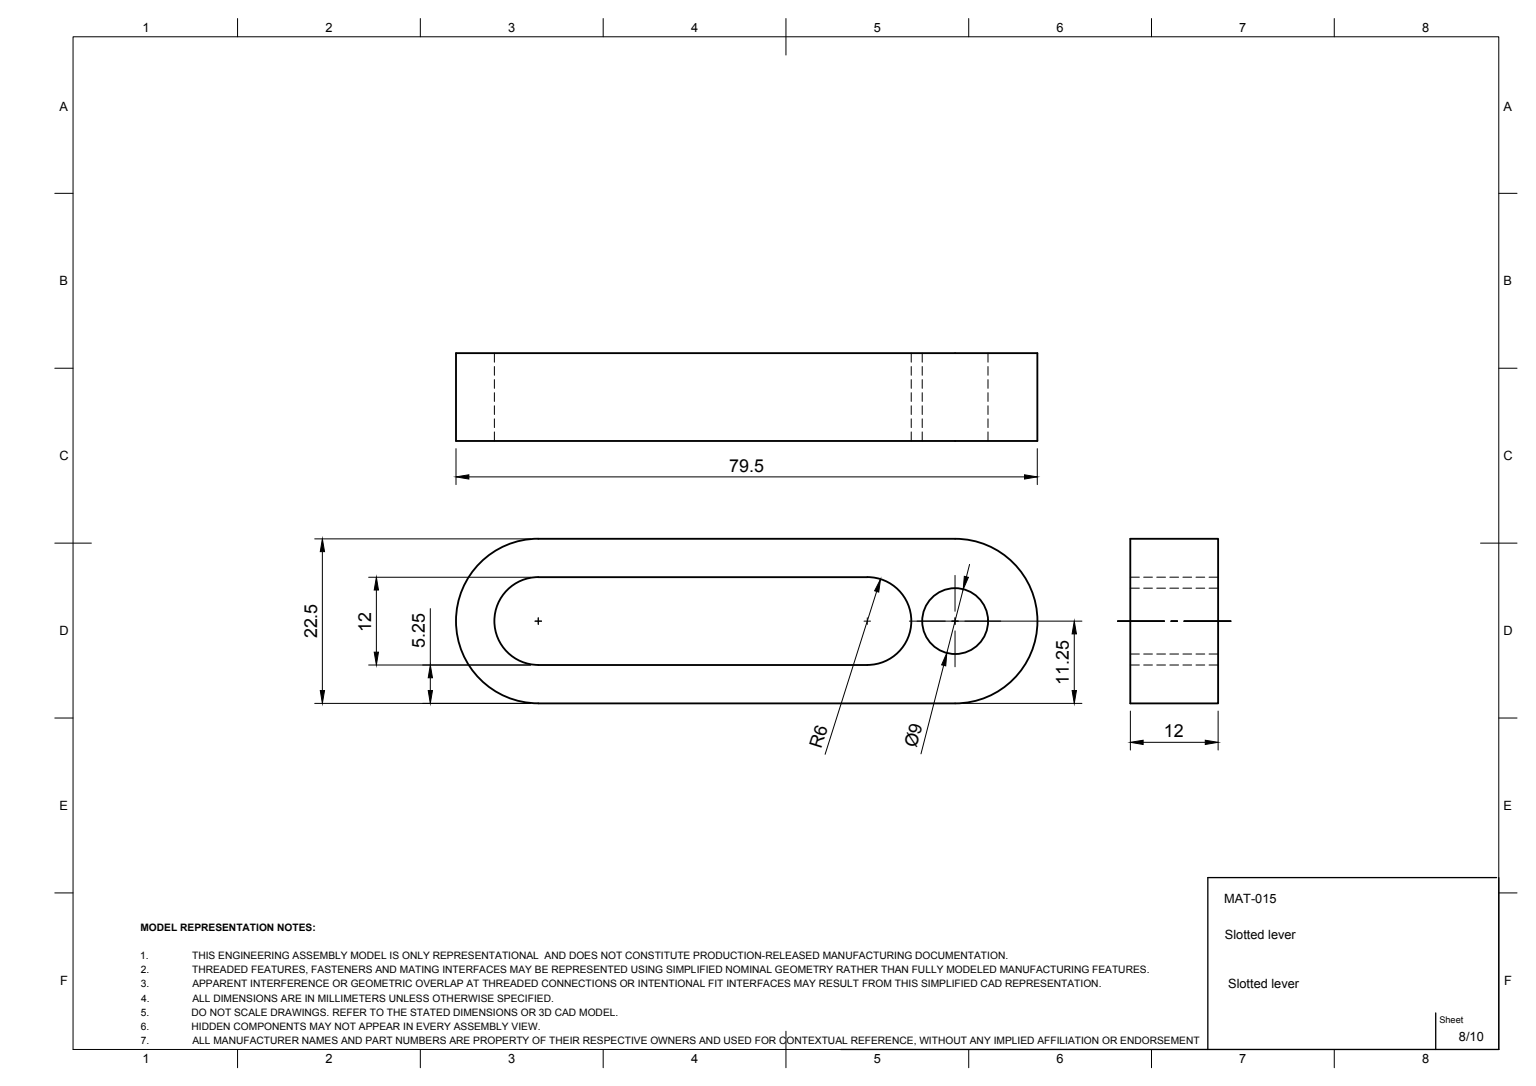
ISO-10303-21;
HEADER;
/* Generated by software containing ST-Developer
 * from STEP Tools, Inc. (www.steptools.com) 
 */

FILE_DESCRIPTION(
/* description */ ('STEP AP214'),
/* implementation_level */ '2;1');

FILE_NAME(
/* name */ 'Slotted Lever.step',
/* time_stamp */ '2026-11-14T06:03:18-08:00',
/* author */ (''),
/* organization */ (''),
/* preprocessor_version */ 'ST-DEVELOPER v20.2',
/* originating_system */ 'Autodesk Translation Framework v15.17.0.0',
/* authorisation */ '');

FILE_SCHEMA (('AUTOMOTIVE_DESIGN { 1 0 10303 214 3 1 1 }'));
ENDSEC;

DATA;
#10=MECHANICAL_DESIGN_GEOMETRIC_PRESENTATION_REPRESENTATION('',(#76),#3206);
#60=SHAPE_REPRESENTATION_RELATIONSHIP('SRR','None',#3243,#68);
#68=ADVANCED_BREP_SHAPE_REPRESENTATION('',(#84),#3202);
#76=STYLED_ITEM('',(#3288),#84);
#84=MANIFOLD_SOLID_BREP('Body1',#1783);
#111=PLANE('',#1971);
#112=PLANE('',#1974);
#113=PLANE('',#1978);
#114=PLANE('',#1979);
#115=PLANE('',#1981);
#116=PLANE('',#1982);
#164=FACE_BOUND('',#675,.T.);
#165=FACE_BOUND('',#676,.T.);
#166=FACE_BOUND('',#678,.T.);
#167=FACE_BOUND('',#679,.T.);
#227=LINE('',#2874,#372);
#228=LINE('',#2877,#373);
#229=LINE('',#2882,#374);
#230=LINE('',#2889,#375);
#231=LINE('',#2892,#376);
#232=LINE('',#2897,#377);
#233=LINE('',#2898,#378);
#234=LINE('',#2902,#379);
#235=LINE('',#2903,#380);
#236=LINE('',#2908,#381);
#237=LINE('',#2909,#382);
#238=LINE('',#2911,#383);
#239=LINE('',#2914,#384);
#240=LINE('',#2916,#385);
#241=LINE('',#2917,#386);
#242=LINE('',#2921,#387);
#243=LINE('',#2922,#388);
#372=VECTOR('',#2290,1000.);
#373=VECTOR('',#2293,1000.);
#374=VECTOR('',#2298,4.5);
#375=VECTOR('',#2305,1000.);
#376=VECTOR('',#2308,1000.);
#377=VECTOR('',#2313,1000.);
#378=VECTOR('',#2314,1000.);
#379=VECTOR('',#2317,1000.);
#380=VECTOR('',#2318,1000.);
#381=VECTOR('',#2323,1000.);
#382=VECTOR('',#2324,1000.);
#383=VECTOR('',#2325,1000.);
#384=VECTOR('',#2328,1000.);
#385=VECTOR('',#2331,1000.);
#386=VECTOR('',#2332,1000.);
#387=VECTOR('',#2339,1000.);
#388=VECTOR('',#2340,1000.);
#492=CYLINDRICAL_SURFACE('',#1962,6.);
#493=CYLINDRICAL_SURFACE('',#1965,4.5);
#494=CYLINDRICAL_SURFACE('',#1968,11.25);
#495=CYLINDRICAL_SURFACE('',#1977,11.25);
#496=CYLINDRICAL_SURFACE('',#1980,6.);
#554=FACE_OUTER_BOUND('',#671,.T.);
#555=FACE_OUTER_BOUND('',#672,.T.);
#556=FACE_OUTER_BOUND('',#673,.T.);
#557=FACE_OUTER_BOUND('',#674,.T.);
#558=FACE_OUTER_BOUND('',#677,.T.);
#559=FACE_OUTER_BOUND('',#680,.T.);
#560=FACE_OUTER_BOUND('',#681,.T.);
#561=FACE_OUTER_BOUND('',#682,.T.);
#562=FACE_OUTER_BOUND('',#683,.T.);
#563=FACE_OUTER_BOUND('',#684,.T.);
#564=FACE_OUTER_BOUND('',#685,.T.);
#671=EDGE_LOOP('',(#1379,#1380,#1381,#1382));
#672=EDGE_LOOP('',(#1383,#1384,#1385,#1386));
#673=EDGE_LOOP('',(#1387,#1388,#1389,#1390));
#674=EDGE_LOOP('',(#1391,#1392,#1393,#1394));
#675=EDGE_LOOP('',(#1395,#1396,#1397,#1398));
#676=EDGE_LOOP('',(#1399));
#677=EDGE_LOOP('',(#1400,#1401,#1402,#1403));
#678=EDGE_LOOP('',(#1404,#1405,#1406,#1407));
#679=EDGE_LOOP('',(#1408));
#680=EDGE_LOOP('',(#1409,#1410,#1411,#1412));
#681=EDGE_LOOP('',(#1413,#1414,#1415,#1416));
#682=EDGE_LOOP('',(#1417,#1418,#1419,#1420));
#683=EDGE_LOOP('',(#1421,#1422,#1423,#1424));
#684=EDGE_LOOP('',(#1425,#1426,#1427,#1428));
#685=EDGE_LOOP('',(#1429,#1430,#1431,#1432));
#791=CIRCLE('',#1963,6.);
#792=CIRCLE('',#1964,6.);
#793=CIRCLE('',#1966,4.5);
#794=CIRCLE('',#1967,4.5);
#795=CIRCLE('',#1969,11.25);
#796=CIRCLE('',#1970,11.25);
#797=CIRCLE('',#1972,11.25);
#798=CIRCLE('',#1973,6.);
#799=CIRCLE('',#1975,11.25);
#800=CIRCLE('',#1976,6.);
#888=VERTEX_POINT('',#2870);
#889=VERTEX_POINT('',#2871);
#890=VERTEX_POINT('',#2873);
#891=VERTEX_POINT('',#2875);
#892=VERTEX_POINT('',#2879);
#893=VERTEX_POINT('',#2881);
#894=VERTEX_POINT('',#2885);
#895=VERTEX_POINT('',#2886);
#896=VERTEX_POINT('',#2888);
#897=VERTEX_POINT('',#2890);
#898=VERTEX_POINT('',#2894);
#899=VERTEX_POINT('',#2895);
#900=VERTEX_POINT('',#2899);
#901=VERTEX_POINT('',#2900);
#902=VERTEX_POINT('',#2905);
#903=VERTEX_POINT('',#2906);
#904=VERTEX_POINT('',#2910);
#905=VERTEX_POINT('',#2912);
#1068=EDGE_CURVE('',#888,#889,#791,.T.);
#1069=EDGE_CURVE('',#889,#890,#227,.T.);
#1070=EDGE_CURVE('',#891,#890,#792,.T.);
#1071=EDGE_CURVE('',#888,#891,#228,.T.);
#1072=EDGE_CURVE('',#892,#892,#793,.T.);
#1073=EDGE_CURVE('',#892,#893,#229,.T.);
#1074=EDGE_CURVE('',#893,#893,#794,.T.);
#1075=EDGE_CURVE('',#894,#895,#795,.T.);
#1076=EDGE_CURVE('',#894,#896,#230,.T.);
#1077=EDGE_CURVE('',#896,#897,#796,.T.);
#1078=EDGE_CURVE('',#895,#897,#231,.T.);
#1079=EDGE_CURVE('',#898,#899,#797,.T.);
#1080=EDGE_CURVE('',#899,#894,#232,.T.);
#1081=EDGE_CURVE('',#895,#898,#233,.T.);
#1082=EDGE_CURVE('',#900,#901,#798,.T.);
#1083=EDGE_CURVE('',#889,#900,#234,.T.);
#1084=EDGE_CURVE('',#901,#888,#235,.T.);
#1085=EDGE_CURVE('',#902,#903,#799,.T.);
#1086=EDGE_CURVE('',#897,#902,#236,.T.);
#1087=EDGE_CURVE('',#903,#896,#237,.T.);
#1088=EDGE_CURVE('',#890,#904,#238,.T.);
#1089=EDGE_CURVE('',#904,#905,#800,.T.);
#1090=EDGE_CURVE('',#905,#891,#239,.T.);
#1091=EDGE_CURVE('',#899,#903,#240,.T.);
#1092=EDGE_CURVE('',#898,#902,#241,.T.);
#1093=EDGE_CURVE('',#900,#904,#242,.T.);
#1094=EDGE_CURVE('',#901,#905,#243,.T.);
#1379=ORIENTED_EDGE('',*,*,#1068,.T.);
#1380=ORIENTED_EDGE('',*,*,#1069,.T.);
#1381=ORIENTED_EDGE('',*,*,#1070,.F.);
#1382=ORIENTED_EDGE('',*,*,#1071,.F.);
#1383=ORIENTED_EDGE('',*,*,#1072,.T.);
#1384=ORIENTED_EDGE('',*,*,#1073,.T.);
#1385=ORIENTED_EDGE('',*,*,#1074,.F.);
#1386=ORIENTED_EDGE('',*,*,#1073,.F.);
#1387=ORIENTED_EDGE('',*,*,#1075,.F.);
#1388=ORIENTED_EDGE('',*,*,#1076,.T.);
#1389=ORIENTED_EDGE('',*,*,#1077,.T.);
#1390=ORIENTED_EDGE('',*,*,#1078,.F.);
#1391=ORIENTED_EDGE('',*,*,#1079,.T.);
#1392=ORIENTED_EDGE('',*,*,#1080,.T.);
#1393=ORIENTED_EDGE('',*,*,#1075,.T.);
#1394=ORIENTED_EDGE('',*,*,#1081,.T.);
#1395=ORIENTED_EDGE('',*,*,#1082,.F.);
#1396=ORIENTED_EDGE('',*,*,#1083,.F.);
#1397=ORIENTED_EDGE('',*,*,#1068,.F.);
#1398=ORIENTED_EDGE('',*,*,#1084,.F.);
#1399=ORIENTED_EDGE('',*,*,#1072,.F.);
#1400=ORIENTED_EDGE('',*,*,#1085,.F.);
#1401=ORIENTED_EDGE('',*,*,#1086,.F.);
#1402=ORIENTED_EDGE('',*,*,#1077,.F.);
#1403=ORIENTED_EDGE('',*,*,#1087,.F.);
#1404=ORIENTED_EDGE('',*,*,#1088,.T.);
#1405=ORIENTED_EDGE('',*,*,#1089,.T.);
#1406=ORIENTED_EDGE('',*,*,#1090,.T.);
#1407=ORIENTED_EDGE('',*,*,#1070,.T.);
#1408=ORIENTED_EDGE('',*,*,#1074,.T.);
#1409=ORIENTED_EDGE('',*,*,#1085,.T.);
#1410=ORIENTED_EDGE('',*,*,#1091,.F.);
#1411=ORIENTED_EDGE('',*,*,#1079,.F.);
#1412=ORIENTED_EDGE('',*,*,#1092,.T.);
#1413=ORIENTED_EDGE('',*,*,#1087,.T.);
#1414=ORIENTED_EDGE('',*,*,#1076,.F.);
#1415=ORIENTED_EDGE('',*,*,#1080,.F.);
#1416=ORIENTED_EDGE('',*,*,#1091,.T.);
#1417=ORIENTED_EDGE('',*,*,#1086,.T.);
#1418=ORIENTED_EDGE('',*,*,#1092,.F.);
#1419=ORIENTED_EDGE('',*,*,#1081,.F.);
#1420=ORIENTED_EDGE('',*,*,#1078,.T.);
#1421=ORIENTED_EDGE('',*,*,#1089,.F.);
#1422=ORIENTED_EDGE('',*,*,#1093,.F.);
#1423=ORIENTED_EDGE('',*,*,#1082,.T.);
#1424=ORIENTED_EDGE('',*,*,#1094,.T.);
#1425=ORIENTED_EDGE('',*,*,#1090,.F.);
#1426=ORIENTED_EDGE('',*,*,#1094,.F.);
#1427=ORIENTED_EDGE('',*,*,#1084,.T.);
#1428=ORIENTED_EDGE('',*,*,#1071,.T.);
#1429=ORIENTED_EDGE('',*,*,#1088,.F.);
#1430=ORIENTED_EDGE('',*,*,#1069,.F.);
#1431=ORIENTED_EDGE('',*,*,#1083,.T.);
#1432=ORIENTED_EDGE('',*,*,#1093,.T.);
#1721=ADVANCED_FACE('',(#554),#492,.F.);
#1722=ADVANCED_FACE('',(#555),#493,.F.);
#1723=ADVANCED_FACE('',(#556),#494,.T.);
#1724=ADVANCED_FACE('',(#557,#164,#165),#111,.F.);
#1725=ADVANCED_FACE('',(#558,#166,#167),#112,.T.);
#1726=ADVANCED_FACE('',(#559),#495,.T.);
#1727=ADVANCED_FACE('',(#560),#113,.F.);
#1728=ADVANCED_FACE('',(#561),#114,.F.);
#1729=ADVANCED_FACE('',(#562),#496,.F.);
#1730=ADVANCED_FACE('',(#563),#115,.T.);
#1731=ADVANCED_FACE('',(#564),#116,.T.);
#1783=CLOSED_SHELL('',(#1721,#1722,#1723,#1724,#1725,#1726,#1727,#1728,
#1729,#1730,#1731));
#1961=AXIS2_PLACEMENT_3D('',#2868,#2284,#2285);
#1962=AXIS2_PLACEMENT_3D('',#2869,#2286,#2287);
#1963=AXIS2_PLACEMENT_3D('',#2872,#2288,#2289);
#1964=AXIS2_PLACEMENT_3D('',#2876,#2291,#2292);
#1965=AXIS2_PLACEMENT_3D('',#2878,#2294,#2295);
#1966=AXIS2_PLACEMENT_3D('',#2880,#2296,#2297);
#1967=AXIS2_PLACEMENT_3D('',#2883,#2299,#2300);
#1968=AXIS2_PLACEMENT_3D('',#2884,#2301,#2302);
#1969=AXIS2_PLACEMENT_3D('',#2887,#2303,#2304);
#1970=AXIS2_PLACEMENT_3D('',#2891,#2306,#2307);
#1971=AXIS2_PLACEMENT_3D('',#2893,#2309,#2310);
#1972=AXIS2_PLACEMENT_3D('',#2896,#2311,#2312);
#1973=AXIS2_PLACEMENT_3D('',#2901,#2315,#2316);
#1974=AXIS2_PLACEMENT_3D('',#2904,#2319,#2320);
#1975=AXIS2_PLACEMENT_3D('',#2907,#2321,#2322);
#1976=AXIS2_PLACEMENT_3D('',#2913,#2326,#2327);
#1977=AXIS2_PLACEMENT_3D('',#2915,#2329,#2330);
#1978=AXIS2_PLACEMENT_3D('',#2918,#2333,#2334);
#1979=AXIS2_PLACEMENT_3D('',#2919,#2335,#2336);
#1980=AXIS2_PLACEMENT_3D('',#2920,#2337,#2338);
#1981=AXIS2_PLACEMENT_3D('',#2923,#2341,#2342);
#1982=AXIS2_PLACEMENT_3D('',#2924,#2343,#2344);
#2284=DIRECTION('axis',(0.,0.,1.));
#2285=DIRECTION('refdir',(1.,0.,0.));
#2286=DIRECTION('center_axis',(-1.15555796663234E-33,0.,-1.));
#2287=DIRECTION('ref_axis',(-1.,0.,1.15555796663234E-33));
#2288=DIRECTION('center_axis',(1.15555796663234E-33,0.,1.));
#2289=DIRECTION('ref_axis',(1.,0.,-1.15555796663234E-33));
#2290=DIRECTION('',(-1.15555796663234E-33,0.,-1.));
#2291=DIRECTION('center_axis',(1.15555796663234E-33,0.,1.));
#2292=DIRECTION('ref_axis',(1.,0.,-1.15555796663234E-33));
#2293=DIRECTION('',(-1.15555796663234E-33,0.,-1.));
#2294=DIRECTION('center_axis',(-1.15555796663234E-33,0.,-1.));
#2295=DIRECTION('ref_axis',(-1.,0.,1.15555796663234E-33));
#2296=DIRECTION('center_axis',(1.15555796663234E-33,0.,1.));
#2297=DIRECTION('ref_axis',(1.,0.,-1.15555796663234E-33));
#2298=DIRECTION('',(-1.15555796663234E-33,0.,-1.));
#2299=DIRECTION('center_axis',(1.15555796663234E-33,0.,1.));
#2300=DIRECTION('ref_axis',(1.,0.,-1.15555796663234E-33));
#2301=DIRECTION('center_axis',(-1.15555796663234E-33,0.,-1.));
#2302=DIRECTION('ref_axis',(-1.,0.,1.15555796663234E-33));
#2303=DIRECTION('center_axis',(1.15555796663234E-33,0.,1.));
#2304=DIRECTION('ref_axis',(1.,0.,-1.15555796663234E-33));
#2305=DIRECTION('',(-1.15555796663234E-33,0.,-1.));
#2306=DIRECTION('center_axis',(1.15555796663234E-33,0.,1.));
#2307=DIRECTION('ref_axis',(1.,0.,-1.15555796663234E-33));
#2308=DIRECTION('',(-1.15555796663234E-33,0.,-1.));
#2309=DIRECTION('center_axis',(1.15555796663234E-33,0.,-1.));
#2310=DIRECTION('ref_axis',(-1.,0.,-1.15555796663234E-33));
#2311=DIRECTION('center_axis',(1.15555796663234E-33,0.,1.));
#2312=DIRECTION('ref_axis',(-1.,0.,1.15555796663234E-33));
#2313=DIRECTION('',(-1.,0.,-1.15555796663234E-33));
#2314=DIRECTION('',(1.,0.,1.15555796663234E-33));
#2315=DIRECTION('center_axis',(1.15555796663234E-33,0.,1.));
#2316=DIRECTION('ref_axis',(1.,0.,-1.15555796663234E-33));
#2317=DIRECTION('',(1.,0.,1.15555796663234E-33));
#2318=DIRECTION('',(-1.,0.,-1.15555796663234E-33));
#2319=DIRECTION('center_axis',(1.15555796663234E-33,0.,-1.));
#2320=DIRECTION('ref_axis',(-1.,0.,-1.15555796663234E-33));
#2321=DIRECTION('center_axis',(1.15555796663234E-33,0.,1.));
#2322=DIRECTION('ref_axis',(-1.,0.,1.15555796663234E-33));
#2323=DIRECTION('',(1.,0.,1.15555796663234E-33));
#2324=DIRECTION('',(-1.,0.,-1.15555796663234E-33));
#2325=DIRECTION('',(1.,0.,1.15555796663234E-33));
#2326=DIRECTION('center_axis',(1.15555796663234E-33,0.,1.));
#2327=DIRECTION('ref_axis',(1.,0.,-1.15555796663234E-33));
#2328=DIRECTION('',(-1.,0.,-1.15555796663234E-33));
#2329=DIRECTION('center_axis',(-1.15555796663234E-33,0.,-1.));
#2330=DIRECTION('ref_axis',(1.,1.22464679914735E-16,-1.15555796663234E-33));
#2331=DIRECTION('',(-1.15555796663234E-33,0.,-1.));
#2332=DIRECTION('',(-1.15555796663234E-33,0.,-1.));
#2333=DIRECTION('center_axis',(0.,-1.,0.));
#2334=DIRECTION('ref_axis',(-1.15555796663234E-33,0.,-1.));
#2335=DIRECTION('center_axis',(0.,1.,0.));
#2336=DIRECTION('ref_axis',(1.15555796663234E-33,0.,1.));
#2337=DIRECTION('center_axis',(-1.15555796663234E-33,0.,-1.));
#2338=DIRECTION('ref_axis',(1.,1.22464679914735E-16,-1.15555796663234E-33));
#2339=DIRECTION('',(-1.15555796663234E-33,0.,-1.));
#2340=DIRECTION('',(-1.15555796663234E-33,0.,-1.));
#2341=DIRECTION('center_axis',(0.,-1.,0.));
#2342=DIRECTION('ref_axis',(-1.15555796663234E-33,0.,-1.));
#2343=DIRECTION('center_axis',(0.,1.,0.));
#2344=DIRECTION('ref_axis',(1.15555796663234E-33,0.,1.));
#2868=CARTESIAN_POINT('',(0.,0.,0.));
#2869=CARTESIAN_POINT('Origin',(3.22849876867702,3.46944695195361E-14,10.));
#2870=CARTESIAN_POINT('',(3.22849876867702,6.00000000000004,10.));
#2871=CARTESIAN_POINT('',(3.22849876867701,-5.99999999999996,10.));
#2872=CARTESIAN_POINT('Origin',(3.22849876867702,3.46944695195361E-14,10.));
#2873=CARTESIAN_POINT('',(3.22849876867702,-5.99999999999996,-2.));
#2874=CARTESIAN_POINT('',(3.22849876867701,-5.99999999999996,10.));
#2875=CARTESIAN_POINT('',(3.22849876867702,6.00000000000004,-2.));
#2876=CARTESIAN_POINT('Origin',(3.22849876867702,3.46944695195361E-14,-2.));
#2877=CARTESIAN_POINT('',(3.22849876867702,6.00000000000004,10.));
#2878=CARTESIAN_POINT('Origin',(-8.77150123132294,0.,10.));
#2879=CARTESIAN_POINT('',(-4.27150123132294,-5.51091059616309E-16,10.));
#2880=CARTESIAN_POINT('Origin',(-8.77150123132294,0.,10.));
#2881=CARTESIAN_POINT('',(-4.27150123132294,-5.51091059616309E-16,-2.));
#2882=CARTESIAN_POINT('',(-4.27150123132294,-5.51091059616309E-16,10.));
#2883=CARTESIAN_POINT('Origin',(-8.77150123132295,0.,-2.));
#2884=CARTESIAN_POINT('Origin',(-8.77150123132294,0.,10.));
#2885=CARTESIAN_POINT('',(-8.77150123132294,11.2500000000001,10.));
#2886=CARTESIAN_POINT('',(-8.77150123132298,-11.25,10.));
#2887=CARTESIAN_POINT('Origin',(-8.77150123132294,0.,10.));
#2888=CARTESIAN_POINT('',(-8.77150123132295,11.2500000000001,-2.));
#2889=CARTESIAN_POINT('',(-8.77150123132294,11.2500000000001,10.));
#2890=CARTESIAN_POINT('',(-8.771501231323,-11.25,-2.));
#2891=CARTESIAN_POINT('Origin',(-8.77150123132295,0.,-2.));
#2892=CARTESIAN_POINT('',(-8.77150123132298,-11.25,10.));
#2893=CARTESIAN_POINT('Origin',(48.228498768677,4.16333634234434E-14,10.));
#2894=CARTESIAN_POINT('',(48.228498768677,-11.25,10.));
#2895=CARTESIAN_POINT('',(48.228498768677,11.25,10.));
#2896=CARTESIAN_POINT('Origin',(48.228498768677,4.16333634234434E-14,10.));
#2897=CARTESIAN_POINT('',(-8.77150123132294,11.2500000000001,10.));
#2898=CARTESIAN_POINT('',(48.228498768677,-11.25,10.));
#2899=CARTESIAN_POINT('',(48.228498768677,-5.99999999999996,10.));
#2900=CARTESIAN_POINT('',(48.228498768677,6.00000000000004,10.));
#2901=CARTESIAN_POINT('Origin',(48.228498768677,4.16333634234434E-14,10.));
#2902=CARTESIAN_POINT('',(48.228498768677,-5.99999999999996,10.));
#2903=CARTESIAN_POINT('',(48.228498768677,6.00000000000004,10.));
#2904=CARTESIAN_POINT('Origin',(48.228498768677,4.16333634234434E-14,-1.99999999999999));
#2905=CARTESIAN_POINT('',(48.228498768677,-11.25,-1.99999999999999));
#2906=CARTESIAN_POINT('',(48.228498768677,11.25,-1.99999999999999));
#2907=CARTESIAN_POINT('Origin',(48.228498768677,4.16333634234434E-14,-1.99999999999999));
#2908=CARTESIAN_POINT('',(48.228498768677,-11.25,-1.99999999999999));
#2909=CARTESIAN_POINT('',(-8.77150123132295,11.2500000000001,-2.));
#2910=CARTESIAN_POINT('',(48.228498768677,-5.99999999999996,-1.99999999999999));
#2911=CARTESIAN_POINT('',(48.228498768677,-5.99999999999996,-1.99999999999999));
#2912=CARTESIAN_POINT('',(48.228498768677,6.00000000000004,-1.99999999999999));
#2913=CARTESIAN_POINT('Origin',(48.228498768677,4.16333634234434E-14,-1.99999999999999));
#2914=CARTESIAN_POINT('',(48.228498768677,6.00000000000004,-1.99999999999999));
#2915=CARTESIAN_POINT('Origin',(48.228498768677,4.16333634234434E-14,10.));
#2916=CARTESIAN_POINT('',(48.228498768677,11.25,10.));
#2917=CARTESIAN_POINT('',(48.228498768677,-11.25,10.));
#2918=CARTESIAN_POINT('Origin',(-8.77150123132294,11.2500000000001,10.));
#2919=CARTESIAN_POINT('Origin',(48.228498768677,-11.25,10.));
#2920=CARTESIAN_POINT('Origin',(48.228498768677,4.16333634234434E-14,10.));
#2921=CARTESIAN_POINT('',(48.228498768677,-5.99999999999996,10.));
#2922=CARTESIAN_POINT('',(48.228498768677,6.00000000000004,10.));
#2923=CARTESIAN_POINT('Origin',(48.228498768677,6.00000000000004,10.));
#2924=CARTESIAN_POINT('Origin',(48.228498768677,-5.99999999999996,10.));
#3192=UNCERTAINTY_MEASURE_WITH_UNIT(LENGTH_MEASURE(0.01),#3207,
'DISTANCE_ACCURACY_VALUE',
'Maximum model space distance between geometric entities at asserted c
onnectivities');
#3196=UNCERTAINTY_MEASURE_WITH_UNIT(LENGTH_MEASURE(0.01),#3207,
'DISTANCE_ACCURACY_VALUE',
'Maximum model space distance between geometric entities at asserted c
onnectivities');
#3202=(
GEOMETRIC_REPRESENTATION_CONTEXT(3)
GLOBAL_UNCERTAINTY_ASSIGNED_CONTEXT((#3192))
GLOBAL_UNIT_ASSIGNED_CONTEXT((#3207,#3209,#3210))
REPRESENTATION_CONTEXT('','3D')
);
#3206=(
GEOMETRIC_REPRESENTATION_CONTEXT(3)
GLOBAL_UNCERTAINTY_ASSIGNED_CONTEXT((#3196))
GLOBAL_UNIT_ASSIGNED_CONTEXT((#3207,#3209,#3210))
REPRESENTATION_CONTEXT('','3D')
);
#3207=(
LENGTH_UNIT()
NAMED_UNIT(*)
SI_UNIT(.MILLI.,.METRE.)
);
#3209=(
NAMED_UNIT(*)
PLANE_ANGLE_UNIT()
SI_UNIT($,.RADIAN.)
);
#3210=(
NAMED_UNIT(*)
SI_UNIT($,.STERADIAN.)
SOLID_ANGLE_UNIT()
);
#3216=SHAPE_DEFINITION_REPRESENTATION(#3225,#3243);
#3225=PRODUCT_DEFINITION_SHAPE('',$,#3253);
#3243=SHAPE_REPRESENTATION('',(#1961),#3202);
#3247=PRODUCT_DEFINITION_CONTEXT('part definition',#3276,'design');
#3253=PRODUCT_DEFINITION('Slotted lever','Slotted Lever',#3262,#3247);
#3262=PRODUCT_DEFINITION_FORMATION('',$,#3283);
#3276=APPLICATION_CONTEXT(
'Core Data for Automotive Mechanical Design Process');
#3277=PRODUCT_CONTEXT('part definition',#3276,'mechanical');
#3283=PRODUCT('Slotted lever','Slotted Lever','Slotted lever',(#3277));
#3288=PRESENTATION_STYLE_ASSIGNMENT((#3292));
#3292=SURFACE_STYLE_USAGE(.BOTH.,#3296);
#3296=SURFACE_SIDE_STYLE('',(#3300));
#3300=SURFACE_STYLE_FILL_AREA(#3304);
#3304=FILL_AREA_STYLE('Opaque(61,176,222)',(#3308));
#3308=FILL_AREA_STYLE_COLOUR('Opaque(61,176,222)',#3312);
#3312=COLOUR_RGB('Opaque(61,176,222)',0.23921568627451,0.690196078431373,
0.870588235294118);
ENDSEC;
END-ISO-10303-21;
